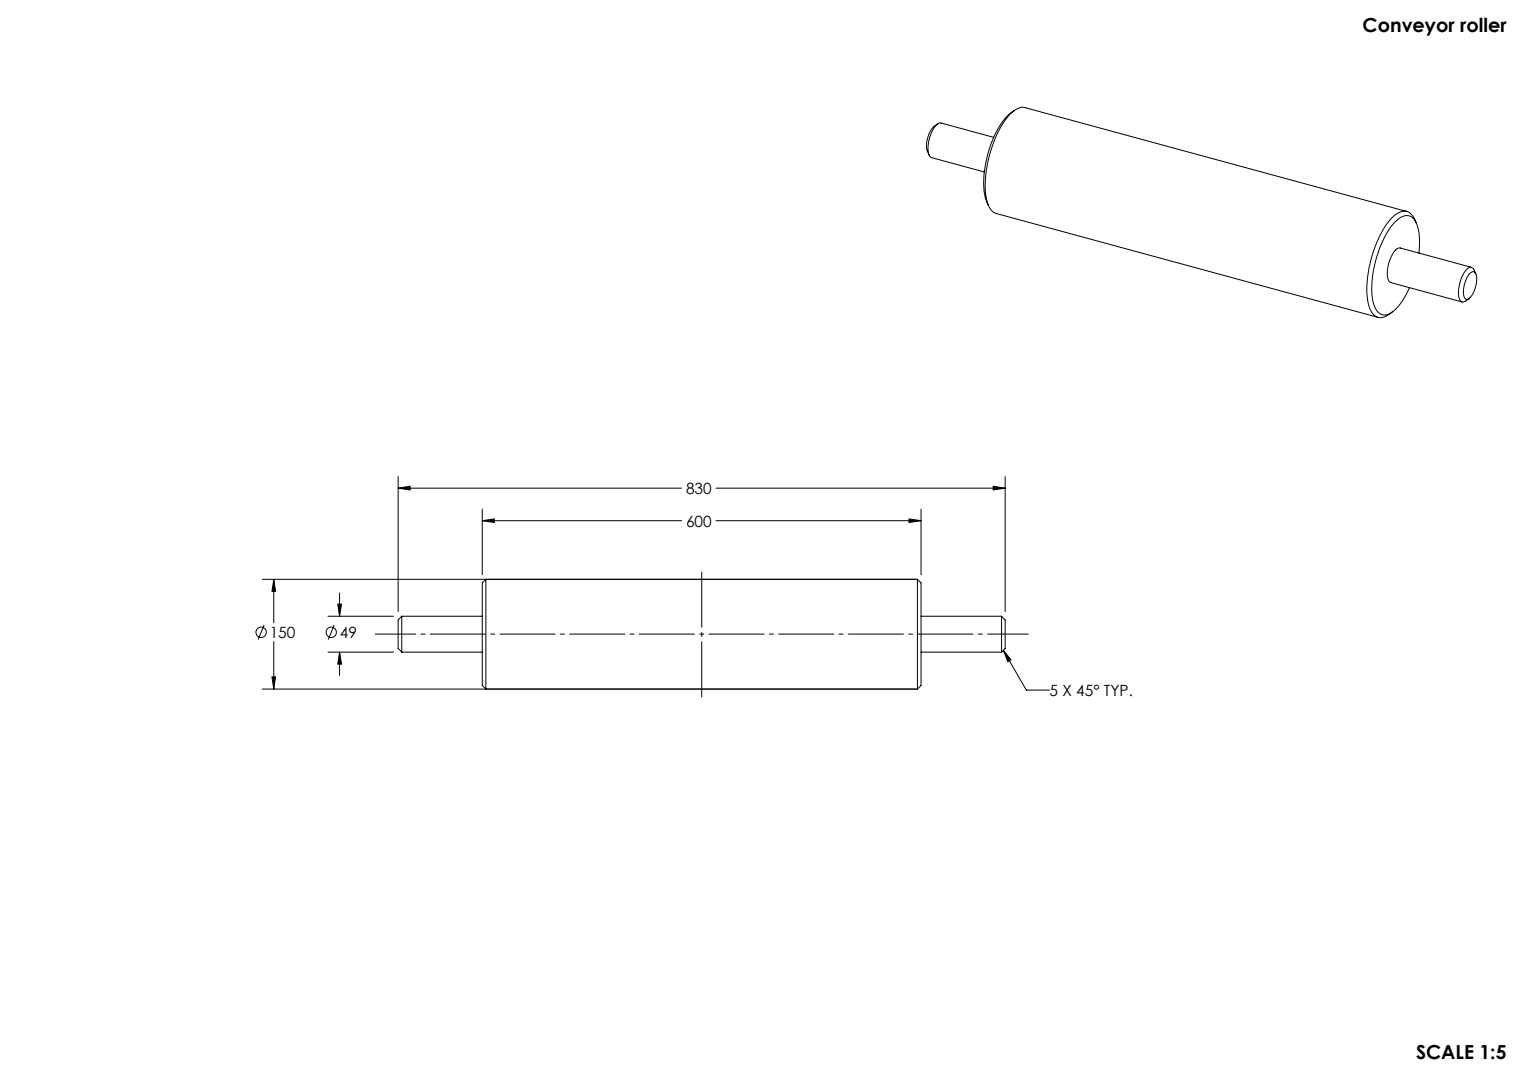
ISO-10303-21;
HEADER;
FILE_DESCRIPTION (('STEP AP214'),
    '1' );
FILE_NAME ('Conveyor roller.step',
    '2026-10-24T15:53:57',
    ( '' ),
    ( '' ),
    'SwSTEP 2.0',
    'SolidWorks 2025',
    '' );
FILE_SCHEMA (( 'AUTOMOTIVE_DESIGN' ));
ENDSEC;

DATA;
#13=DIRECTION ( 'NONE',  ( -1.034996974062501909E-32, 0.7071067811865503483, 0.7071067811865446862 ) ) ;
#29=DIRECTION ( 'NONE',  ( 8.659560562354951347E-17, 0.7071067811865459074, -0.7071067811865491270 ) ) ;
#82=DIRECTION ( 'NONE',  ( -1.463706757734299248E-32, 1.000000000000000000, 5.238529448733281520E-32 ) ) ;
#128=EDGE_LOOP ( 'NONE', ( #8016, #5711, #5284, #7956 ) ) ;
#158=DIRECTION ( 'NONE',  ( 1.463706757734299248E-32, -1.000000000000000000, -5.238529448733281520E-32 ) ) ;
#183=CIRCLE ( 'NONE', #891, 19.49999999999996803 ) ;
#185=ORIENTED_EDGE ( 'NONE', *, *, #1131, .T. ) ;
#239=ORIENTED_EDGE ( 'NONE', *, *, #4179, .F. ) ;
#304=VECTOR ( 'NONE', #6582, 1000.000000000000114 ) ;
#309=CARTESIAN_POINT ( 'NONE',  ( 3.000384657911014680E-15, -299.9999999999999432, -24.50000000000001776 ) ) ;
#323=DIRECTION ( 'NONE',  ( 1.463706757734299248E-32, -1.000000000000000000, -5.238529448733281520E-32 ) ) ;
#343=EDGE_CURVE ( 'NONE', #1391, #6892, #2509, .T. ) ;
#344=DIRECTION ( 'NONE',  ( -1.463706757734299248E-32, 1.000000000000000000, 5.238529448733281520E-32 ) ) ;
#347=EDGE_LOOP ( 'NONE', ( #894, #7668, #7763, #5691 ) ) ;
#369=VERTEX_POINT ( 'NONE', #3034 ) ;
#386=EDGE_CURVE ( 'NONE', #7541, #369, #1275, .T. ) ;
#460=CYLINDRICAL_SURFACE ( 'NONE', #6966, 75.00000000000005684 ) ;
#480=CONICAL_SURFACE ( 'NONE', #3807, 75.00000000000005684, 0.7853981633974441712 ) ;
#482=DIRECTION ( 'NONE',  ( 1.463706757734299248E-32, -1.000000000000000000, -5.238529448733281520E-32 ) ) ;
#490=DIRECTION ( 'NONE',  ( 0.000000000000000000, 0.000000000000000000, -1.000000000000000000 ) ) ;
#513=( LENGTH_UNIT ( ) NAMED_UNIT ( * ) SI_UNIT ( .MILLI., .METRE. ) );
#524=CARTESIAN_POINT ( 'NONE',  ( 0.000000000000000000, -294.9999999999998295, -2.775557561562891351E-14 ) ) ;
#538=EDGE_LOOP ( 'NONE', ( #1198, #7491, #4676, #8222 ) ) ;
#564=LINE ( 'NONE', #5822, #7147 ) ;
#577=FACE_OUTER_BOUND ( 'NONE', #538, .T. ) ;
#599=CIRCLE ( 'NONE', #8258, 70.00000000000008527 ) ;
#603=CARTESIAN_POINT ( 'NONE',  ( 0.000000000000000000, -294.9999999999998295, 75.00000000000002842 ) ) ;
#640=EDGE_LOOP ( 'NONE', ( #7745, #1073, #1566, #6105 ) ) ;
#653=EDGE_CURVE ( 'NONE', #369, #7541, #599, .T. ) ;
#656=FACE_OUTER_BOUND ( 'NONE', #3276, .T. ) ;
#668=DIRECTION ( 'NONE',  ( 1.463706757734299248E-32, -1.000000000000000000, -5.238529448733281520E-32 ) ) ;
#689=CIRCLE ( 'NONE', #1791, 19.49999999999996803 ) ;
#707=MECHANICAL_DESIGN_GEOMETRIC_PRESENTATION_REPRESENTATION('',(#5446),#1666);
#732=EDGE_CURVE ( 'NONE', #3003, #1200, #8389, .T. ) ;
#736=ORIENTED_EDGE ( 'NONE', *, *, #8068, .T. ) ;
#746=CIRCLE ( 'NONE', #5638, 19.49999999999996803 ) ;
#769=EDGE_CURVE ( 'NONE', #6892, #1241, #3931, .T. ) ;
#779=FACE_OUTER_BOUND ( 'NONE', #7734, .T. ) ;
#786=EDGE_CURVE ( 'NONE', #1663, #7888, #746, .T. ) ;
#798=DIRECTION ( 'NONE',  ( 0.000000000000000000, 0.000000000000000000, 1.000000000000000000 ) ) ;
#830=AXIS2_PLACEMENT_3D ( 'NONE', #5763, #4510, #5888 ) ;
#837=DIRECTION ( 'NONE',  ( 0.000000000000000000, 0.000000000000000000, 1.000000000000000000 ) ) ;
#884=CYLINDRICAL_SURFACE ( 'NONE', #4494, 24.50000000000000000 ) ;
#891=AXIS2_PLACEMENT_3D ( 'NONE', #3001, #5687, #2958 ) ;
#894=ORIENTED_EDGE ( 'NONE', *, *, #7114, .T. ) ;
#957=CARTESIAN_POINT ( 'NONE',  ( 0.000000000000000000, -299.9999999999999432, 75.00000000000002842 ) ) ;
#972=EDGE_CURVE ( 'NONE', #1241, #5649, #1680, .T. ) ;
#978=DIRECTION ( 'NONE',  ( 1.034996974062501909E-32, -0.7071067811865503483, -0.7071067811865446862 ) ) ;
#980=CIRCLE ( 'NONE', #3190, 24.49999999999999645 ) ;
#991=( NAMED_UNIT ( * ) SI_UNIT ( $, .STERADIAN. ) SOLID_ANGLE_UNIT ( ) );
#1015=EDGE_CURVE ( 'NONE', #8125, #3237, #183, .T. ) ;
#1073=ORIENTED_EDGE ( 'NONE', *, *, #5836, .F. ) ;
#1095=ORIENTED_EDGE ( 'NONE', *, *, #386, .F. ) ;
#1096=DIRECTION ( 'NONE',  ( -1.463706757734299248E-32, 1.000000000000000000, 5.238529448733281520E-32 ) ) ;
#1101=AXIS2_PLACEMENT_3D ( 'NONE', #2723, #668, #4640 ) ;
#1112=ADVANCED_FACE ( 'NONE', ( #7873 ), #2726, .T. ) ;
#1120=CARTESIAN_POINT ( 'NONE',  ( 3.659266894335830776E-32, -299.9999999999999432, 69.99999999999992895 ) ) ;
#1131=EDGE_CURVE ( 'NONE', #5665, #6135, #2302, .T. ) ;
#1135=ORIENTED_EDGE ( 'NONE', *, *, #343, .T. ) ;
#1144=DIRECTION ( 'NONE',  ( -1.463706757734299248E-32, 1.000000000000000000, 5.238529448733281520E-32 ) ) ;
#1150=ORIENTED_EDGE ( 'NONE', *, *, #5995, .F. ) ;
#1172=DIRECTION ( 'NONE',  ( 1.463706757734299248E-32, -1.000000000000000000, 4.930380657631321594E-32 ) ) ;
#1198=ORIENTED_EDGE ( 'NONE', *, *, #1015, .F. ) ;
#1200=VERTEX_POINT ( 'NONE', #5219 ) ;
#1204=ADVANCED_FACE ( 'NONE', ( #7784 ), #1471, .T. ) ;
#1232=ADVANCED_FACE ( 'NONE', ( #779, #7221 ), #4563, .F. ) ;
#1241=VERTEX_POINT ( 'NONE', #3296 ) ;
#1275=CIRCLE ( 'NONE', #3368, 70.00000000000008527 ) ;
#1277=CIRCLE ( 'NONE', #4765, 24.50000000000000000 ) ;
#1331=CARTESIAN_POINT ( 'NONE',  ( 3.000384657911015074E-15, -299.9999999999999432, -24.50000000000002487 ) ) ;
#1366=CARTESIAN_POINT ( 'NONE',  ( 3.000384657910866768E-15, -410.0000000000000568, -24.50000000000005684 ) ) ;
#1391=VERTEX_POINT ( 'NONE', #7613 ) ;
#1412=DIRECTION ( 'NONE',  ( -1.463706757734299248E-32, 1.000000000000000000, 5.238529448733281520E-32 ) ) ;
#1420=DIRECTION ( 'NONE',  ( -1.463706757734299248E-32, 1.000000000000000000, 5.238529448733281520E-32 ) ) ;
#1422=LINE ( 'NONE', #2550, #7952 ) ;
#1440=CARTESIAN_POINT ( 'NONE',  ( 0.000000000000000000, 415.0000000000000000, -19.50000000000002487 ) ) ;
#1441=DIRECTION ( 'NONE',  ( -1.463706757734299248E-32, 1.000000000000000000, 5.238529448733281520E-32 ) ) ;
#1457=AXIS2_PLACEMENT_3D ( 'NONE', #3998, #158, #5980 ) ;
#1471=CONICAL_SURFACE ( 'NONE', #6621, 70.00000000000008527, 0.7853981633974441712 ) ;
#1483=ORIENTED_EDGE ( 'NONE', *, *, #6085, .F. ) ;
#1490=CYLINDRICAL_SURFACE ( 'NONE', #5481, 24.49999999999999645 ) ;
#1528=FACE_OUTER_BOUND ( 'NONE', #347, .T. ) ;
#1537=ORIENTED_EDGE ( 'NONE', *, *, #4179, .T. ) ;
#1540=DIRECTION ( 'NONE',  ( 0.000000000000000000, 0.000000000000000000, 1.000000000000000000 ) ) ;
#1553=CYLINDRICAL_SURFACE ( 'NONE', #8324, 24.50000000000000000 ) ;
#1566=ORIENTED_EDGE ( 'NONE', *, *, #4780, .T. ) ;
#1603=EDGE_CURVE ( 'NONE', #3424, #7090, #8161, .T. ) ;
#1618=FACE_OUTER_BOUND ( 'NONE', #7265, .T. ) ;
#1649=DIRECTION ( 'NONE',  ( 0.000000000000000000, 0.000000000000000000, 1.000000000000000000 ) ) ;
#1651=LINE ( 'NONE', #7798, #7932 ) ;
#1658=ORIENTED_EDGE ( 'NONE', *, *, #3292, .F. ) ;
#1663=VERTEX_POINT ( 'NONE', #6553 ) ;
#1666=( GEOMETRIC_REPRESENTATION_CONTEXT ( 3 ) GLOBAL_UNCERTAINTY_ASSIGNED_CONTEXT ( ( #3671 ) ) GLOBAL_UNIT_ASSIGNED_CONTEXT ( ( #513, #1770, #7866 ) ) REPRESENTATION_CONTEXT ( 'NONE', 'WORKASPACE' ) );
#1671=DIRECTION ( 'NONE',  ( 1.463706757734299248E-32, -1.000000000000000000, -5.238529448733281520E-32 ) ) ;
#1679=EDGE_LOOP ( 'NONE', ( #2046, #5402, #7077, #4475 ) ) ;
#1680=LINE ( 'NONE', #957, #5485 ) ;
#1684=ORIENTED_EDGE ( 'NONE', *, *, #2466, .F. ) ;
#1688=CARTESIAN_POINT ( 'NONE',  ( 3.000384657911015074E-15, -299.9999999999999432, -24.50000000000002842 ) ) ;
#1690=AXIS2_PLACEMENT_3D ( 'NONE', #3227, #5915, #8579 ) ;
#1699=LINE ( 'NONE', #7593, #3623 ) ;
#1725=EDGE_LOOP ( 'NONE', ( #736, #8188 ) ) ;
#1756=CARTESIAN_POINT ( 'NONE',  ( 3.000384657911007580E-15, 410.0000000000000000, -24.50000000000004619 ) ) ;
#1770=( NAMED_UNIT ( * ) PLANE_ANGLE_UNIT ( ) SI_UNIT ( $, .RADIAN. ) );
#1771=EDGE_LOOP ( 'NONE', ( #185, #4295 ) ) ;
#1791=AXIS2_PLACEMENT_3D ( 'NONE', #3676, #7068, #5743 ) ;
#1800=ORIENTED_EDGE ( 'NONE', *, *, #653, .F. ) ;
#1832=VECTOR ( 'NONE', #7210, 1000.000000000000114 ) ;
#1839=CARTESIAN_POINT ( 'NONE',  ( 0.000000000000000000, -299.9999999999999432, -2.775557561562891351E-14 ) ) ;
#1851=DIRECTION ( 'NONE',  ( -1.463706757734299248E-32, 1.000000000000000000, 5.238529448733281520E-32 ) ) ;
#1863=LINE ( 'NONE', #603, #7517 ) ;
#1900=AXIS2_PLACEMENT_3D ( 'NONE', #3813, #1671, #2374 ) ;
#1911=DIRECTION ( 'NONE',  ( -1.463706757734299248E-32, 1.000000000000000000, 5.238529448733281520E-32 ) ) ;
#1934=CARTESIAN_POINT ( 'NONE',  ( 1.355854680848614041E-28, -410.0000000000000568, 24.49999999999991829 ) ) ;
#1961=AXIS2_PLACEMENT_3D ( 'NONE', #4989, #5805, #8467 ) ;
#1985=LINE ( 'NONE', #3333, #7711 ) ;
#1988=CARTESIAN_POINT ( 'NONE',  ( 1.110223024625156540E-13, -414.9999999999999432, -4.163336342344337027E-14 ) ) ;
#1996=( GEOMETRIC_REPRESENTATION_CONTEXT ( 3 ) GLOBAL_UNCERTAINTY_ASSIGNED_CONTEXT ( ( #4363 ) ) GLOBAL_UNIT_ASSIGNED_CONTEXT ( ( #6312, #8302, #991 ) ) REPRESENTATION_CONTEXT ( 'NONE', 'WORKASPACE' ) );
#2018=CARTESIAN_POINT ( 'NONE',  ( 0.000000000000000000, 415.0000000000000000, -5.551115123125782702E-14 ) ) ;
#2027=LINE ( 'NONE', #1331, #3362 ) ;
#2046=ORIENTED_EDGE ( 'NONE', *, *, #786, .F. ) ;
#2086=CARTESIAN_POINT ( 'NONE',  ( 0.000000000000000000, 299.9999999999999432, -5.551115123125782702E-14 ) ) ;
#2139=AXIS2_PLACEMENT_3D ( 'NONE', #4194, #2201, #4850 ) ;
#2159=DIRECTION ( 'NONE',  ( 0.000000000000000000, 0.000000000000000000, 1.000000000000000000 ) ) ;
#2172=FACE_OUTER_BOUND ( 'NONE', #7634, .T. ) ;
#2199=CYLINDRICAL_SURFACE ( 'NONE', #8478, 24.49999999999999645 ) ;
#2201=DIRECTION ( 'NONE',  ( 1.463706757734299248E-32, -1.000000000000000000, -5.238529448733281520E-32 ) ) ;
#2219=LINE ( 'NONE', #3527, #4211 ) ;
#2247=CYLINDRICAL_SURFACE ( 'NONE', #8107, 75.00000000000005684 ) ;
#2294=ADVANCED_FACE ( 'NONE', ( #2312 ), #7081, .T. ) ;
#2302=CIRCLE ( 'NONE', #5667, 24.50000000000000000 ) ;
#2312=FACE_OUTER_BOUND ( 'NONE', #640, .T. ) ;
#2318=PLANE ( 'NONE',  #3189 ) ;
#2327=FACE_OUTER_BOUND ( 'NONE', #8408, .T. ) ;
#2345=APPLICATION_CONTEXT ( 'automotive_design' ) ;
#2347=DIRECTION ( 'NONE',  ( 0.000000000000000000, 0.000000000000000000, -1.000000000000000000 ) ) ;
#2350=CIRCLE ( 'NONE', #6531, 69.99999999999998579 ) ;
#2351=CARTESIAN_POINT ( 'NONE',  ( 2.694222958124174048E-15, 415.0000000000000000, 19.49999999999990763 ) ) ;
#2374=DIRECTION ( 'NONE',  ( 0.000000000000000000, 0.000000000000000000, -1.000000000000000000 ) ) ;
#2384=CARTESIAN_POINT ( 'NONE',  ( 0.000000000000000000, 299.9999999999999432, -6.938893903907228378E-14 ) ) ;
#2408=ADVANCED_FACE ( 'NONE', ( #577 ), #7504, .T. ) ;
#2413=CARTESIAN_POINT ( 'NONE',  ( 1.110223024625156540E-13, -410.0000000000000568, -6.938893903907228378E-14 ) ) ;
#2431=ADVANCED_FACE ( 'NONE', ( #3932 ), #4730, .T. ) ;
#2452=DIRECTION ( 'NONE',  ( -4.440892098500626951E-15, 0.000000000000000000, -1.000000000000000000 ) ) ;
#2466=EDGE_CURVE ( 'NONE', #1391, #5417, #2350, .T. ) ;
#2509=LINE ( 'NONE', #4553, #1832 ) ;
#2520=DIRECTION ( 'NONE',  ( 0.000000000000000000, 0.000000000000000000, -1.000000000000000000 ) ) ;
#2536=SHAPE_REPRESENTATION ( 'Conveyor roller', ( #7563 ), #1996 ) ;
#2550=CARTESIAN_POINT ( 'NONE',  ( 9.184850993605156622E-15, -299.9999999999999432, -75.00000000000008527 ) ) ;
#2580=PRODUCT_CONTEXT ( 'NONE', #2345, 'mechanical' ) ;
#2592=DIRECTION ( 'NONE',  ( -1.463706757734299248E-32, 1.000000000000000000, 5.238529448733281520E-32 ) ) ;
#2628=CONICAL_SURFACE ( 'NONE', #830, 24.49999999999999645, 0.7853981633974503884 ) ;
#2668=DIRECTION ( 'NONE',  ( 0.000000000000000000, 0.000000000000000000, 1.000000000000000000 ) ) ;
#2692=CARTESIAN_POINT ( 'NONE',  ( 0.000000000000000000, 299.9999999999999432, 24.49999999999994316 ) ) ;
#2694=DIRECTION ( 'NONE',  ( 0.000000000000000000, 0.000000000000000000, -1.000000000000000000 ) ) ;
#2695=DIRECTION ( 'NONE',  ( 1.463706757734299248E-32, -1.000000000000000000, 4.930380657631321594E-32 ) ) ;
#2723=CARTESIAN_POINT ( 'NONE',  ( 0.000000000000000000, 299.9999999999999432, -6.938893903907228378E-14 ) ) ;
#2726=CONICAL_SURFACE ( 'NONE', #3269, 19.49999999999996803, 0.7853981633974507215 ) ;
#2785=ORIENTED_EDGE ( 'NONE', *, *, #8184, .T. ) ;
#2877=AXIS2_PLACEMENT_3D ( 'NONE', #7868, #8603, #2694 ) ;
#2911=VECTOR ( 'NONE', #1096, 1000.000000000000000 ) ;
#2925=DIRECTION ( 'NONE',  ( -1.463706757734299248E-32, 1.000000000000000000, 5.238529448733281520E-32 ) ) ;
#2929=CARTESIAN_POINT ( 'NONE',  ( 1.110223024625156540E-13, -414.9999999999999432, 19.49999999999989342 ) ) ;
#2943=DIRECTION ( 'NONE',  ( -1.463706757734299248E-32, 1.000000000000000000, 5.238529448733281520E-32 ) ) ;
#2946=MANIFOLD_SOLID_BREP ( 'Chamfer1', #4312 ) ;
#2958=DIRECTION ( 'NONE',  ( 0.000000000000000000, 0.000000000000000000, -1.000000000000000000 ) ) ;
#2974=ADVANCED_FACE ( 'NONE', ( #4083 ), #6065, .T. ) ;
#2983=CARTESIAN_POINT ( 'NONE',  ( 1.110223024625156540E-13, -414.9999999999999432, -6.938893903907228378E-14 ) ) ;
#3001=CARTESIAN_POINT ( 'NONE',  ( 0.000000000000000000, 415.0000000000000000, -5.551115123125782702E-14 ) ) ;
#3003=VERTEX_POINT ( 'NONE', #2692 ) ;
#3012=LINE ( 'NONE', #7112, #2911 ) ;
#3021=ORIENTED_EDGE ( 'NONE', *, *, #769, .T. ) ;
#3034=CARTESIAN_POINT ( 'NONE',  ( 0.000000000000000000, 299.9999999999999432, -70.00000000000015632 ) ) ;
#3061=ADVANCED_FACE ( 'NONE', ( #2327 ), #2247, .T. ) ;
#3090=LINE ( 'NONE', #1688, #6449 ) ;
#3094=ORIENTED_EDGE ( 'NONE', *, *, #5793, .T. ) ;
#3138=CARTESIAN_POINT ( 'NONE',  ( 1.110223024625156540E-13, -410.0000000000000568, -6.938893903907228378E-14 ) ) ;
#3171=DIRECTION ( 'NONE',  ( -1.463706757734299248E-32, 1.000000000000000000, 5.238529448733281520E-32 ) ) ;
#3189=AXIS2_PLACEMENT_3D ( 'NONE', #4974, #2695, #3385 ) ;
#3190=AXIS2_PLACEMENT_3D ( 'NONE', #2413, #8300, #2452 ) ;
#3223=CARTESIAN_POINT ( 'NONE',  ( 0.000000000000000000, -294.9999999999998295, -2.775557561562891351E-14 ) ) ;
#3227=CARTESIAN_POINT ( 'NONE',  ( 0.000000000000000000, -299.9999999999999432, -2.775557561562891351E-14 ) ) ;
#3237=VERTEX_POINT ( 'NONE', #1440 ) ;
#3269=AXIS2_PLACEMENT_3D ( 'NONE', #3787, #5733, #7019 ) ;
#3276=EDGE_LOOP ( 'NONE', ( #4309, #7256, #3094, #7788 ) ) ;
#3292=EDGE_CURVE ( 'NONE', #7541, #5649, #2219, .T. ) ;
#3296=CARTESIAN_POINT ( 'NONE',  ( -4.391120273202897044E-30, -294.9999999999998295, 75.00000000000000000 ) ) ;
#3307=DIRECTION ( 'NONE',  ( 0.000000000000000000, -4.930380657631321594E-32, -1.000000000000000000 ) ) ;
#3318=CIRCLE ( 'NONE', #5723, 75.00000000000005684 ) ;
#3323=ORIENTED_EDGE ( 'NONE', *, *, #6119, .F. ) ;
#3327=CARTESIAN_POINT ( 'NONE',  ( 0.000000000000000000, 299.9999999999999432, -6.938893903907228378E-14 ) ) ;
#3333=CARTESIAN_POINT ( 'NONE',  ( 0.000000000000000000, -299.9999999999999432, 24.49999999999996803 ) ) ;
#3352=DIRECTION ( 'NONE',  ( 0.000000000000000000, 0.000000000000000000, 1.000000000000000000 ) ) ;
#3362=VECTOR ( 'NONE', #6554, 1000.000000000000000 ) ;
#3368=AXIS2_PLACEMENT_3D ( 'NONE', #6435, #7127, #8436 ) ;
#3381=CIRCLE ( 'NONE', #2139, 75.00000000000005684 ) ;
#3384=FACE_OUTER_BOUND ( 'NONE', #8499, .T. ) ;
#3385=DIRECTION ( 'NONE',  ( 0.000000000000000000, -4.930380657631321594E-32, -1.000000000000000000 ) ) ;
#3413=VERTEX_POINT ( 'NONE', #1934 ) ;
#3424=VERTEX_POINT ( 'NONE', #1756 ) ;
#3463=ORIENTED_EDGE ( 'NONE', *, *, #8095, .F. ) ;
#3493=AXIS2_PLACEMENT_3D ( 'NONE', #1988, #6749, #7955 ) ;
#3512=DIRECTION ( 'NONE',  ( 1.000000000000000000, 0.000000000000000000, 0.000000000000000000 ) ) ;
#3527=CARTESIAN_POINT ( 'NONE',  ( 8.572527594031484037E-15, 299.9999999999999432, 70.00000000000001421 ) ) ;
#3551=DIRECTION ( 'NONE',  ( -1.463706757734299248E-32, 1.000000000000000000, 5.238529448733281520E-32 ) ) ;
#3577=ADVANCED_BREP_SHAPE_REPRESENTATION ( '', ( #2946, #7563 ), #1996 ) ;
#3580=DIRECTION ( 'NONE',  ( -1.463706757734299248E-32, 1.000000000000000000, 5.238529448733281520E-32 ) ) ;
#3613=AXIS2_PLACEMENT_3D ( 'NONE', #3138, #6417, #1649 ) ;
#3623=VECTOR ( 'NONE', #978, 1000.000000000000114 ) ;
#3625=ORIENTED_EDGE ( 'NONE', *, *, #1603, .T. ) ;
#3632=EDGE_CURVE ( 'NONE', #6135, #5665, #5470, .T. ) ;
#3648=SHAPE_REPRESENTATION_RELATIONSHIP ( 'NONE' , 'NONE' ,  #2536, #3577 ) ;
#3671=UNCERTAINTY_MEASURE_WITH_UNIT (LENGTH_MEASURE( 1.000000000000000082E-05 ), #513, 'distance_accuracy_value', 'NONE');
#3676=CARTESIAN_POINT ( 'NONE',  ( 0.000000000000000000, 415.0000000000000000, -5.551115123125782702E-14 ) ) ;
#3701=APPLICATION_CONTEXT ( 'automotive_design' ) ;
#3703=ORIENTED_EDGE ( 'NONE', *, *, #972, .F. ) ;
#3787=CARTESIAN_POINT ( 'NONE',  ( 0.000000000000000000, 415.0000000000000000, -5.551115123125782702E-14 ) ) ;
#3807=AXIS2_PLACEMENT_3D ( 'NONE', #6577, #1441, #3352 ) ;
#3812=CARTESIAN_POINT ( 'NONE',  ( 0.000000000000000000, 299.9999999999999432, -6.938893903907228378E-14 ) ) ;
#3813=CARTESIAN_POINT ( 'NONE',  ( 0.000000000000000000, 410.0000000000000000, -5.551115123125782702E-14 ) ) ;
#3822=CIRCLE ( 'NONE', #1457, 69.99999999999998579 ) ;
#3852=FACE_OUTER_BOUND ( 'NONE', #1679, .T. ) ;
#3872=CIRCLE ( 'NONE', #5562, 24.49999999999999645 ) ;
#3927=ORIENTED_EDGE ( 'NONE', *, *, #6427, .F. ) ;
#3931=CIRCLE ( 'NONE', #7560, 75.00000000000005684 ) ;
#3932=FACE_OUTER_BOUND ( 'NONE', #6566, .T. ) ;
#3996=DIRECTION ( 'NONE',  ( 1.463706757734299248E-32, -1.000000000000000000, 4.930380657631321594E-32 ) ) ;
#3998=CARTESIAN_POINT ( 'NONE',  ( 0.000000000000000000, -299.9999999999999432, -2.775557561562891351E-14 ) ) ;
#3999=ORIENTED_EDGE ( 'NONE', *, *, #8040, .T. ) ;
#4070=ORIENTED_EDGE ( 'NONE', *, *, #3632, .F. ) ;
#4083=FACE_OUTER_BOUND ( 'NONE', #7475, .T. ) ;
#4140=DIRECTION ( 'NONE',  ( -1.463706757734299248E-32, 1.000000000000000000, 5.238529448733281520E-32 ) ) ;
#4150=ORIENTED_EDGE ( 'NONE', *, *, #653, .T. ) ;
#4169=CARTESIAN_POINT ( 'NONE',  ( 0.000000000000000000, -299.9999999999999432, -2.775557561562891351E-14 ) ) ;
#4179=EDGE_CURVE ( 'NONE', #8044, #5649, #3381, .T. ) ;
#4192=CARTESIAN_POINT ( 'NONE',  ( 0.000000000000000000, -299.9999999999999432, -2.775557561562891351E-14 ) ) ;
#4194=CARTESIAN_POINT ( 'NONE',  ( 0.000000000000000000, 295.0000000000000568, -6.938893903907228378E-14 ) ) ;
#4199=ORIENTED_EDGE ( 'NONE', *, *, #7570, .T. ) ;
#4203=CARTESIAN_POINT ( 'NONE',  ( 0.000000000000000000, 0.000000000000000000, 0.000000000000000000 ) ) ;
#4211=VECTOR ( 'NONE', #6202, 1000.000000000000114 ) ;
#4236=FACE_OUTER_BOUND ( 'NONE', #7497, .T. ) ;
#4279=DIRECTION ( 'NONE',  ( 1.463706757734299248E-32, -1.000000000000000000, -5.238529448733281520E-32 ) ) ;
#4282=FACE_BOUND ( 'NONE', #1771, .T. ) ;
#4293=DIRECTION ( 'NONE',  ( 0.000000000000000000, 0.000000000000000000, 1.000000000000000000 ) ) ;
#4295=ORIENTED_EDGE ( 'NONE', *, *, #3632, .T. ) ;
#4309=ORIENTED_EDGE ( 'NONE', *, *, #343, .F. ) ;
#4312=CLOSED_SHELL ( 'NONE', ( #1204, #2408, #7124, #6395, #3061, #4564, #4579, #7024, #2974, #5264, #5278, #7558, #1232, #4790, #4403, #2294, #1112, #2431 ) ) ;
#4326=DIRECTION ( 'NONE',  ( 1.034996974062495067E-32, -0.7071067811865456854, -0.7071067811865493491 ) ) ;
#4363=UNCERTAINTY_MEASURE_WITH_UNIT (LENGTH_MEASURE( 1.000000000000000082E-05 ), #6312, 'distance_accuracy_value', 'NONE');
#4379=PRODUCT_DEFINITION_FORMATION_WITH_SPECIFIED_SOURCE ( 'ANY', '', #6615, .NOT_KNOWN. ) ;
#4403=ADVANCED_FACE ( 'NONE', ( #656 ), #480, .T. ) ;
#4470=ORIENTED_EDGE ( 'NONE', *, *, #386, .T. ) ;
#4475=ORIENTED_EDGE ( 'NONE', *, *, #4780, .F. ) ;
#4483=DIRECTION ( 'NONE',  ( -1.463706757734299248E-32, 1.000000000000000000, 5.238529448733281520E-32 ) ) ;
#4485=LINE ( 'NONE', #5230, #304 ) ;
#4494=AXIS2_PLACEMENT_3D ( 'NONE', #6086, #82, #798 ) ;
#4510=DIRECTION ( 'NONE',  ( -1.463706757734299248E-32, 1.000000000000000000, 5.238529448733281520E-32 ) ) ;
#4553=CARTESIAN_POINT ( 'NONE',  ( 9.184850993605156622E-15, -294.9999999999998295, -75.00000000000008527 ) ) ;
#4563=PLANE ( 'NONE',  #5671 ) ;
#4564=ADVANCED_FACE ( 'NONE', ( #1528 ), #1490, .T. ) ;
#4572=EDGE_LOOP ( 'NONE', ( #1684, #1135, #4681, #8189 ) ) ;
#4579=ADVANCED_FACE ( 'NONE', ( #4236 ), #884, .T. ) ;
#4640=DIRECTION ( 'NONE',  ( 0.000000000000000000, 0.000000000000000000, -1.000000000000000000 ) ) ;
#4670=FACE_OUTER_BOUND ( 'NONE', #1725, .T. ) ;
#4676=ORIENTED_EDGE ( 'NONE', *, *, #1603, .F. ) ;
#4681=ORIENTED_EDGE ( 'NONE', *, *, #6764, .F. ) ;
#4686=ORIENTED_EDGE ( 'NONE', *, *, #5995, .T. ) ;
#4717=EDGE_CURVE ( 'NONE', #1200, #3424, #3090, .T. ) ;
#4730=CONICAL_SURFACE ( 'NONE', #1101, 70.00000000000008527, 0.7853981633974441712 ) ;
#4765=AXIS2_PLACEMENT_3D ( 'NONE', #6743, #5600, #2347 ) ;
#4780=EDGE_CURVE ( 'NONE', #7888, #3413, #564, .T. ) ;
#4790=ADVANCED_FACE ( 'NONE', ( #4670 ), #5951, .F. ) ;
#4812=DIRECTION ( 'NONE',  ( 0.000000000000000000, 0.000000000000000000, -1.000000000000000000 ) ) ;
#4850=DIRECTION ( 'NONE',  ( 0.000000000000000000, 0.000000000000000000, -1.000000000000000000 ) ) ;
#4878=CIRCLE ( 'NONE', #1961, 19.49999999999996803 ) ;
#4911=CARTESIAN_POINT ( 'NONE',  ( -9.587279263159650267E-30, 410.0000000000000000, 24.49999999999993605 ) ) ;
#4961=EDGE_CURVE ( 'NONE', #1663, #7727, #6806, .T. ) ;
#4974=CARTESIAN_POINT ( 'NONE',  ( 0.000000000000000000, -299.9999999999999432, 0.000000000000000000 ) ) ;
#4989=CARTESIAN_POINT ( 'NONE',  ( 1.110223024625156540E-13, -414.9999999999999432, -6.938893903907228378E-14 ) ) ;
#5052=EDGE_CURVE ( 'NONE', #5649, #8044, #6376, .T. ) ;
#5134=EDGE_LOOP ( 'NONE', ( #6016, #3927 ) ) ;
#5192=AXIS2_PLACEMENT_3D ( 'NONE', #7149, #1172, #3307 ) ;
#5219=CARTESIAN_POINT ( 'NONE',  ( 3.000384657911011130E-15, 299.9999999999999432, -24.50000000000007461 ) ) ;
#5230=CARTESIAN_POINT ( 'NONE',  ( 2.388061258337334995E-15, 415.0000000000000000, 19.49999999999991473 ) ) ;
#5252=EDGE_CURVE ( 'NONE', #369, #8044, #1699, .T. ) ;
#5264=ADVANCED_FACE ( 'NONE', ( #3384 ), #2199, .T. ) ;
#5278=ADVANCED_FACE ( 'NONE', ( #1618, #4282 ), #2318, .T. ) ;
#5284=ORIENTED_EDGE ( 'NONE', *, *, #8095, .T. ) ;
#5312=ORIENTED_EDGE ( 'NONE', *, *, #2466, .T. ) ;
#5368=CARTESIAN_POINT ( 'NONE',  ( 0.000000000000000000, 299.9999999999999432, -6.938893903907228378E-14 ) ) ;
#5402=ORIENTED_EDGE ( 'NONE', *, *, #4961, .T. ) ;
#5417=VERTEX_POINT ( 'NONE', #1120 ) ;
#5446=STYLED_ITEM('',(#8677),#2946);
#5470=CIRCLE ( 'NONE', #1690, 24.50000000000000000 ) ;
#5481=AXIS2_PLACEMENT_3D ( 'NONE', #7369, #1412, #2159 ) ;
#5485=VECTOR ( 'NONE', #3580, 1000.000000000000000 ) ;
#5562=AXIS2_PLACEMENT_3D ( 'NONE', #5844, #1851, #7087 ) ;
#5600=DIRECTION ( 'NONE',  ( 1.463706757734299248E-32, -1.000000000000000000, -5.238529448733281520E-32 ) ) ;
#5613=ORIENTED_EDGE ( 'NONE', *, *, #5836, .T. ) ;
#5638=AXIS2_PLACEMENT_3D ( 'NONE', #2983, #323, #490 ) ;
#5649=VERTEX_POINT ( 'NONE', #5933 ) ;
#5657=ORIENTED_EDGE ( 'NONE', *, *, #4717, .T. ) ;
#5665=VERTEX_POINT ( 'NONE', #5974 ) ;
#5667=AXIS2_PLACEMENT_3D ( 'NONE', #5813, #3171, #7096 ) ;
#5671=AXIS2_PLACEMENT_3D ( 'NONE', #2086, #3996, #5977 ) ;
#5677=DIRECTION ( 'NONE',  ( 0.000000000000000000, 0.000000000000000000, 1.000000000000000000 ) ) ;
#5687=DIRECTION ( 'NONE',  ( -1.463706757734299248E-32, 1.000000000000000000, 5.238529448733281520E-32 ) ) ;
#5691=ORIENTED_EDGE ( 'NONE', *, *, #7291, .F. ) ;
#5711=ORIENTED_EDGE ( 'NONE', *, *, #6427, .T. ) ;
#5723=AXIS2_PLACEMENT_3D ( 'NONE', #5814, #1911, #6570 ) ;
#5733=DIRECTION ( 'NONE',  ( 1.463706757734299248E-32, -1.000000000000000000, -5.238529448733281520E-32 ) ) ;
#5743=DIRECTION ( 'NONE',  ( 0.000000000000000000, 0.000000000000000000, -1.000000000000000000 ) ) ;
#5763=CARTESIAN_POINT ( 'NONE',  ( 1.110223024625156540E-13, -410.0000000000000568, -6.938893903907228378E-14 ) ) ;
#5793=EDGE_CURVE ( 'NONE', #5417, #1241, #1863, .T. ) ;
#5805=DIRECTION ( 'NONE',  ( 1.463706757734299248E-32, -1.000000000000000000, -5.238529448733281520E-32 ) ) ;
#5813=CARTESIAN_POINT ( 'NONE',  ( 0.000000000000000000, -299.9999999999999432, -2.775557561562891351E-14 ) ) ;
#5814=CARTESIAN_POINT ( 'NONE',  ( 0.000000000000000000, -294.9999999999998295, -2.775557561562891351E-14 ) ) ;
#5822=CARTESIAN_POINT ( 'NONE',  ( 1.110223024625156540E-13, -410.0000000000000568, 24.49999999999992895 ) ) ;
#5836=EDGE_CURVE ( 'NONE', #7888, #1663, #4878, .T. ) ;
#5844=CARTESIAN_POINT ( 'NONE',  ( 1.110223024625156540E-13, -410.0000000000000568, -6.938893903907228378E-14 ) ) ;
#5888=DIRECTION ( 'NONE',  ( 0.000000000000000000, 0.000000000000000000, 1.000000000000000000 ) ) ;
#5915=DIRECTION ( 'NONE',  ( -1.463706757734299248E-32, 1.000000000000000000, 5.238529448733281520E-32 ) ) ;
#5932=DIRECTION ( 'NONE',  ( -1.463706757734299248E-32, 1.000000000000000000, 5.238529448733281520E-32 ) ) ;
#5933=CARTESIAN_POINT ( 'NONE',  ( -4.391120273202894942E-30, 295.0000000000000568, 74.99999999999995737 ) ) ;
#5951=PLANE ( 'NONE',  #5192 ) ;
#5974=CARTESIAN_POINT ( 'NONE',  ( 0.000000000000000000, -299.9999999999999432, 24.49999999999997158 ) ) ;
#5977=DIRECTION ( 'NONE',  ( 0.000000000000000000, -4.930380657631321594E-32, -1.000000000000000000 ) ) ;
#5980=DIRECTION ( 'NONE',  ( 0.000000000000000000, 0.000000000000000000, -1.000000000000000000 ) ) ;
#5986=ORIENTED_EDGE ( 'NONE', *, *, #5252, .F. ) ;
#5995=EDGE_CURVE ( 'NONE', #6892, #8044, #1422, .T. ) ;
#6016=ORIENTED_EDGE ( 'NONE', *, *, #732, .F. ) ;
#6032=CARTESIAN_POINT ( 'NONE',  ( 1.140226871204266778E-13, -410.0000000000000568, -24.50000000000006750 ) ) ;
#6039=SHAPE_DEFINITION_REPRESENTATION ( #6772, #2536 ) ;
#6041=CIRCLE ( 'NONE', #7553, 24.50000000000001066 ) ;
#6065=PLANE ( 'NONE',  #3493 ) ;
#6085=EDGE_CURVE ( 'NONE', #7727, #6135, #2027, .T. ) ;
#6086=CARTESIAN_POINT ( 'NONE',  ( 0.000000000000000000, -299.9999999999999432, -2.775557561562891351E-14 ) ) ;
#6105=ORIENTED_EDGE ( 'NONE', *, *, #7570, .F. ) ;
#6119=EDGE_CURVE ( 'NONE', #7090, #3424, #1277, .T. ) ;
#6135=VERTEX_POINT ( 'NONE', #309 ) ;
#6147=ORIENTED_EDGE ( 'NONE', *, *, #5052, .T. ) ;
#6202=DIRECTION ( 'NONE',  ( 8.659560562354899578E-17, -0.7071067811865503483, 0.7071067811865446862 ) ) ;
#6220=DIRECTION ( 'NONE',  ( 0.000000000000000000, 0.000000000000000000, 1.000000000000000000 ) ) ;
#6251=EDGE_CURVE ( 'NONE', #8125, #7090, #4485, .T. ) ;
#6253=EDGE_LOOP ( 'NONE', ( #8338, #6793, #3999, #3323 ) ) ;
#6301=CARTESIAN_POINT ( 'NONE',  ( 0.000000000000000000, -299.9999999999999432, -2.775557561562891351E-14 ) ) ;
#6312=( LENGTH_UNIT ( ) NAMED_UNIT ( * ) SI_UNIT ( .MILLI., .METRE. ) );
#6349=ORIENTED_EDGE ( 'NONE', *, *, #5052, .F. ) ;
#6360=DIRECTION ( 'NONE',  ( 0.000000000000000000, 0.000000000000000000, -1.000000000000000000 ) ) ;
#6376=CIRCLE ( 'NONE', #2877, 75.00000000000005684 ) ;
#6395=ADVANCED_FACE ( 'NONE', ( #7839 ), #7822, .T. ) ;
#6417=DIRECTION ( 'NONE',  ( -1.463706757734299248E-32, 1.000000000000000000, 5.238529448733281520E-32 ) ) ;
#6427=EDGE_CURVE ( 'NONE', #1200, #3003, #6041, .T. ) ;
#6435=CARTESIAN_POINT ( 'NONE',  ( 0.000000000000000000, 299.9999999999999432, -6.938893903907228378E-14 ) ) ;
#6449=VECTOR ( 'NONE', #2925, 1000.000000000000000 ) ;
#6468=DIRECTION ( 'NONE',  ( -1.463706757734299248E-32, 1.000000000000000000, 5.238529448733281520E-32 ) ) ;
#6531=AXIS2_PLACEMENT_3D ( 'NONE', #6301, #4279, #4812 ) ;
#6553=CARTESIAN_POINT ( 'NONE',  ( 1.137165254206398273E-13, -414.9999999999999432, -19.50000000000003197 ) ) ;
#6554=DIRECTION ( 'NONE',  ( -1.463706757734299248E-32, 1.000000000000000000, 5.238529448733281520E-32 ) ) ;
#6557=ORIENTED_EDGE ( 'NONE', *, *, #3292, .T. ) ;
#6566=EDGE_LOOP ( 'NONE', ( #1658, #1800, #8451, #6349 ) ) ;
#6570=DIRECTION ( 'NONE',  ( 0.000000000000000000, 0.000000000000000000, -1.000000000000000000 ) ) ;
#6577=CARTESIAN_POINT ( 'NONE',  ( 0.000000000000000000, -294.9999999999998295, -2.775557561562891351E-14 ) ) ;
#6580=AXIS2_PLACEMENT_3D ( 'NONE', #3223, #4140, #2668 ) ;
#6582=DIRECTION ( 'NONE',  ( 8.659560562354956277E-17, -0.7071067811865456854, 0.7071067811865493491 ) ) ;
#6615=PRODUCT ( 'Conveyor roller', 'Conveyor roller', '', ( #2580 ) ) ;
#6621=AXIS2_PLACEMENT_3D ( 'NONE', #2384, #482, #2520 ) ;
#6682=ORIENTED_EDGE ( 'NONE', *, *, #6764, .T. ) ;
#6731=DIRECTION ( 'NONE',  ( 0.000000000000000000, 0.000000000000000000, -1.000000000000000000 ) ) ;
#6743=CARTESIAN_POINT ( 'NONE',  ( 0.000000000000000000, 410.0000000000000000, -5.551115123125782702E-14 ) ) ;
#6749=DIRECTION ( 'NONE',  ( 1.463706757734299248E-32, -1.000000000000000000, 4.930380657631321594E-32 ) ) ;
#6764=EDGE_CURVE ( 'NONE', #1241, #6892, #3318, .T. ) ;
#6772=PRODUCT_DEFINITION_SHAPE ( 'NONE', 'NONE',  #8285 ) ;
#6789=VECTOR ( 'NONE', #29, 1000.000000000000114 ) ;
#6793=ORIENTED_EDGE ( 'NONE', *, *, #8068, .F. ) ;
#6806=LINE ( 'NONE', #6032, #6789 ) ;
#6808=DIRECTION ( 'NONE',  ( -1.463706757734299248E-32, 1.000000000000000000, 5.238529448733281520E-32 ) ) ;
#6892=VERTEX_POINT ( 'NONE', #8049 ) ;
#6966=AXIS2_PLACEMENT_3D ( 'NONE', #1839, #1144, #7001 ) ;
#7001=DIRECTION ( 'NONE',  ( 0.000000000000000000, 0.000000000000000000, 1.000000000000000000 ) ) ;
#7019=DIRECTION ( 'NONE',  ( 0.000000000000000000, 0.000000000000000000, -1.000000000000000000 ) ) ;
#7024=ADVANCED_FACE ( 'NONE', ( #8311 ), #1553, .T. ) ;
#7068=DIRECTION ( 'NONE',  ( -1.463706757734299248E-32, 1.000000000000000000, 5.238529448733281520E-32 ) ) ;
#7077=ORIENTED_EDGE ( 'NONE', *, *, #7114, .F. ) ;
#7081=CONICAL_SURFACE ( 'NONE', #3613, 24.49999999999999645, 0.7853981633974503884 ) ;
#7087=DIRECTION ( 'NONE',  ( 5.329070518200751394E-15, 0.000000000000000000, -1.000000000000000000 ) ) ;
#7090=VERTEX_POINT ( 'NONE', #4911 ) ;
#7096=DIRECTION ( 'NONE',  ( 0.000000000000000000, 0.000000000000000000, 1.000000000000000000 ) ) ;
#7110=ORIENTED_EDGE ( 'NONE', *, *, #972, .T. ) ;
#7112=CARTESIAN_POINT ( 'NONE',  ( 0.000000000000000000, -299.9999999999999432, 24.49999999999997158 ) ) ;
#7114=EDGE_CURVE ( 'NONE', #3413, #7727, #3872, .T. ) ;
#7124=ADVANCED_FACE ( 'NONE', ( #3852 ), #2628, .T. ) ;
#7127=DIRECTION ( 'NONE',  ( -1.463706757734299248E-32, 1.000000000000000000, 5.238529448733281520E-32 ) ) ;
#7147=VECTOR ( 'NONE', #8448, 1000.000000000000114 ) ;
#7149=CARTESIAN_POINT ( 'NONE',  ( 0.000000000000000000, 415.0000000000000000, -4.163336342344337027E-14 ) ) ;
#7210=DIRECTION ( 'NONE',  ( 8.659560562354897113E-17, 0.7071067811865503483, -0.7071067811865446862 ) ) ;
#7221=FACE_BOUND ( 'NONE', #5134, .T. ) ;
#7236=ORIENTED_EDGE ( 'NONE', *, *, #732, .T. ) ;
#7242=ORIENTED_EDGE ( 'NONE', *, *, #786, .T. ) ;
#7256=ORIENTED_EDGE ( 'NONE', *, *, #8184, .F. ) ;
#7265=EDGE_LOOP ( 'NONE', ( #2785, #5312 ) ) ;
#7291=EDGE_CURVE ( 'NONE', #3413, #5665, #1985, .T. ) ;
#7369=CARTESIAN_POINT ( 'NONE',  ( 0.000000000000000000, -299.9999999999999432, -2.775557561562891351E-14 ) ) ;
#7475=EDGE_LOOP ( 'NONE', ( #5613, #7242 ) ) ;
#7476=CARTESIAN_POINT ( 'NONE',  ( 8.878689293818315596E-15, 299.9999999999999432, 69.99999999999998579 ) ) ;
#7478=DIRECTION ( 'NONE',  ( 0.000000000000000000, 0.000000000000000000, 1.000000000000000000 ) ) ;
#7491=ORIENTED_EDGE ( 'NONE', *, *, #6251, .T. ) ;
#7497=EDGE_LOOP ( 'NONE', ( #7236, #5657, #3625, #3463 ) ) ;
#7503=EDGE_LOOP ( 'NONE', ( #1095, #6557, #239, #5986 ) ) ;
#7504=CONICAL_SURFACE ( 'NONE', #7778, 19.49999999999996803, 0.7853981633974507215 ) ;
#7517=VECTOR ( 'NONE', #13, 1000.000000000000114 ) ;
#7541=VERTEX_POINT ( 'NONE', #7476 ) ;
#7553=AXIS2_PLACEMENT_3D ( 'NONE', #5368, #6808, #837 ) ;
#7558=ADVANCED_FACE ( 'NONE', ( #2172 ), #460, .T. ) ;
#7560=AXIS2_PLACEMENT_3D ( 'NONE', #524, #4483, #7598 ) ;
#7563=AXIS2_PLACEMENT_3D ( 'NONE', #4203, #7478, #3512 ) ;
#7564=CARTESIAN_POINT ( 'NONE',  ( 0.000000000000000000, -299.9999999999999432, -2.775557561562891351E-14 ) ) ;
#7570=EDGE_CURVE ( 'NONE', #7727, #3413, #980, .T. ) ;
#7593=CARTESIAN_POINT ( 'NONE',  ( 0.000000000000000000, 299.9999999999999432, -70.00000000000015632 ) ) ;
#7598=DIRECTION ( 'NONE',  ( 0.000000000000000000, 0.000000000000000000, -1.000000000000000000 ) ) ;
#7613=CARTESIAN_POINT ( 'NONE',  ( 8.878689293818307707E-15, -299.9999999999999432, -69.99999999999998579 ) ) ;
#7634=EDGE_LOOP ( 'NONE', ( #1150, #3021, #7110, #6147 ) ) ;
#7668=ORIENTED_EDGE ( 'NONE', *, *, #6085, .T. ) ;
#7711=VECTOR ( 'NONE', #5932, 1000.000000000000000 ) ;
#7727=VERTEX_POINT ( 'NONE', #1366 ) ;
#7734=EDGE_LOOP ( 'NONE', ( #4150, #4470 ) ) ;
#7745=ORIENTED_EDGE ( 'NONE', *, *, #4961, .F. ) ;
#7763=ORIENTED_EDGE ( 'NONE', *, *, #1131, .F. ) ;
#7778=AXIS2_PLACEMENT_3D ( 'NONE', #2018, #7941, #6731 ) ;
#7784=FACE_OUTER_BOUND ( 'NONE', #7503, .T. ) ;
#7788=ORIENTED_EDGE ( 'NONE', *, *, #769, .F. ) ;
#7798=CARTESIAN_POINT ( 'NONE',  ( 0.000000000000000000, 415.0000000000000000, -19.50000000000002487 ) ) ;
#7822=CONICAL_SURFACE ( 'NONE', #6580, 75.00000000000005684, 0.7853981633974441712 ) ;
#7830=AXIS2_PLACEMENT_3D ( 'NONE', #3327, #1420, #1540 ) ;
#7839=FACE_OUTER_BOUND ( 'NONE', #4572, .T. ) ;
#7857=PRODUCT_DEFINITION_CONTEXT ( 'detailed design', #3701, 'design' ) ;
#7866=( NAMED_UNIT ( * ) SI_UNIT ( $, .STERADIAN. ) SOLID_ANGLE_UNIT ( ) );
#7868=CARTESIAN_POINT ( 'NONE',  ( 0.000000000000000000, 295.0000000000000568, -6.938893903907228378E-14 ) ) ;
#7873=FACE_OUTER_BOUND ( 'NONE', #6253, .T. ) ;
#7888=VERTEX_POINT ( 'NONE', #2929 ) ;
#7932=VECTOR ( 'NONE', #4326, 1000.000000000000114 ) ;
#7941=DIRECTION ( 'NONE',  ( 1.463706757734299248E-32, -1.000000000000000000, -5.238529448733281520E-32 ) ) ;
#7952=VECTOR ( 'NONE', #2592, 1000.000000000000000 ) ;
#7955=DIRECTION ( 'NONE',  ( 0.000000000000000000, -4.930380657631321594E-32, -1.000000000000000000 ) ) ;
#7956=ORIENTED_EDGE ( 'NONE', *, *, #6119, .T. ) ;
#8016=ORIENTED_EDGE ( 'NONE', *, *, #4717, .F. ) ;
#8040=EDGE_CURVE ( 'NONE', #3237, #3424, #1651, .T. ) ;
#8044=VERTEX_POINT ( 'NONE', #8420 ) ;
#8049=CARTESIAN_POINT ( 'NONE',  ( 9.184850993605148733E-15, -294.9999999999998295, -75.00000000000005684 ) ) ;
#8053=ORIENTED_EDGE ( 'NONE', *, *, #7291, .T. ) ;
#8068=EDGE_CURVE ( 'NONE', #3237, #8125, #689, .T. ) ;
#8095=EDGE_CURVE ( 'NONE', #3003, #7090, #3012, .T. ) ;
#8107=AXIS2_PLACEMENT_3D ( 'NONE', #7564, #2943, #4293 ) ;
#8125=VERTEX_POINT ( 'NONE', #2351 ) ;
#8161=CIRCLE ( 'NONE', #1900, 24.50000000000000000 ) ;
#8184=EDGE_CURVE ( 'NONE', #5417, #1391, #3822, .T. ) ;
#8188=ORIENTED_EDGE ( 'NONE', *, *, #1015, .T. ) ;
#8189=ORIENTED_EDGE ( 'NONE', *, *, #5793, .F. ) ;
#8222=ORIENTED_EDGE ( 'NONE', *, *, #8040, .F. ) ;
#8258=AXIS2_PLACEMENT_3D ( 'NONE', #3812, #6468, #6360 ) ;
#8285=PRODUCT_DEFINITION ( 'UNKNOWN', '', #4379, #7857 ) ;
#8300=DIRECTION ( 'NONE',  ( -1.463706757734299248E-32, 1.000000000000000000, 5.238529448733281520E-32 ) ) ;
#8302=( NAMED_UNIT ( * ) PLANE_ANGLE_UNIT ( ) SI_UNIT ( $, .RADIAN. ) );
#8311=FACE_OUTER_BOUND ( 'NONE', #128, .T. ) ;
#8324=AXIS2_PLACEMENT_3D ( 'NONE', #4169, #344, #5677 ) ;
#8338=ORIENTED_EDGE ( 'NONE', *, *, #6251, .F. ) ;
#8389=CIRCLE ( 'NONE', #7830, 24.50000000000001066 ) ;
#8408=EDGE_LOOP ( 'NONE', ( #6682, #4686, #1537, #3703 ) ) ;
#8420=CARTESIAN_POINT ( 'NONE',  ( 9.184850993605153466E-15, 295.0000000000000568, -75.00000000000009948 ) ) ;
#8436=DIRECTION ( 'NONE',  ( 0.000000000000000000, 0.000000000000000000, -1.000000000000000000 ) ) ;
#8448=DIRECTION ( 'NONE',  ( -1.034996974062495478E-32, 0.7071067811865459074, 0.7071067811865491270 ) ) ;
#8451=ORIENTED_EDGE ( 'NONE', *, *, #5252, .T. ) ;
#8467=DIRECTION ( 'NONE',  ( 0.000000000000000000, 0.000000000000000000, -1.000000000000000000 ) ) ;
#8478=AXIS2_PLACEMENT_3D ( 'NONE', #4192, #3551, #6220 ) ;
#8499=EDGE_LOOP ( 'NONE', ( #1483, #4199, #8053, #4070 ) ) ;
#8579=DIRECTION ( 'NONE',  ( 0.000000000000000000, 0.000000000000000000, 1.000000000000000000 ) ) ;
#8603=DIRECTION ( 'NONE',  ( 1.463706757734299248E-32, -1.000000000000000000, -5.238529448733281520E-32 ) ) ;
#8671=COLOUR_RGB('Off White',0.89,0.88,0.83);
#8672=FILL_AREA_STYLE_COLOUR('',#8671);
#8673=FILL_AREA_STYLE('',(#8672));
#8674=SURFACE_STYLE_FILL_AREA(#8673);
#8675=SURFACE_SIDE_STYLE('',(#8674));
#8676=SURFACE_STYLE_USAGE(.BOTH.,#8675);
#8677=PRESENTATION_STYLE_ASSIGNMENT((#8676));
ENDSEC;
END-ISO-10303-21;
